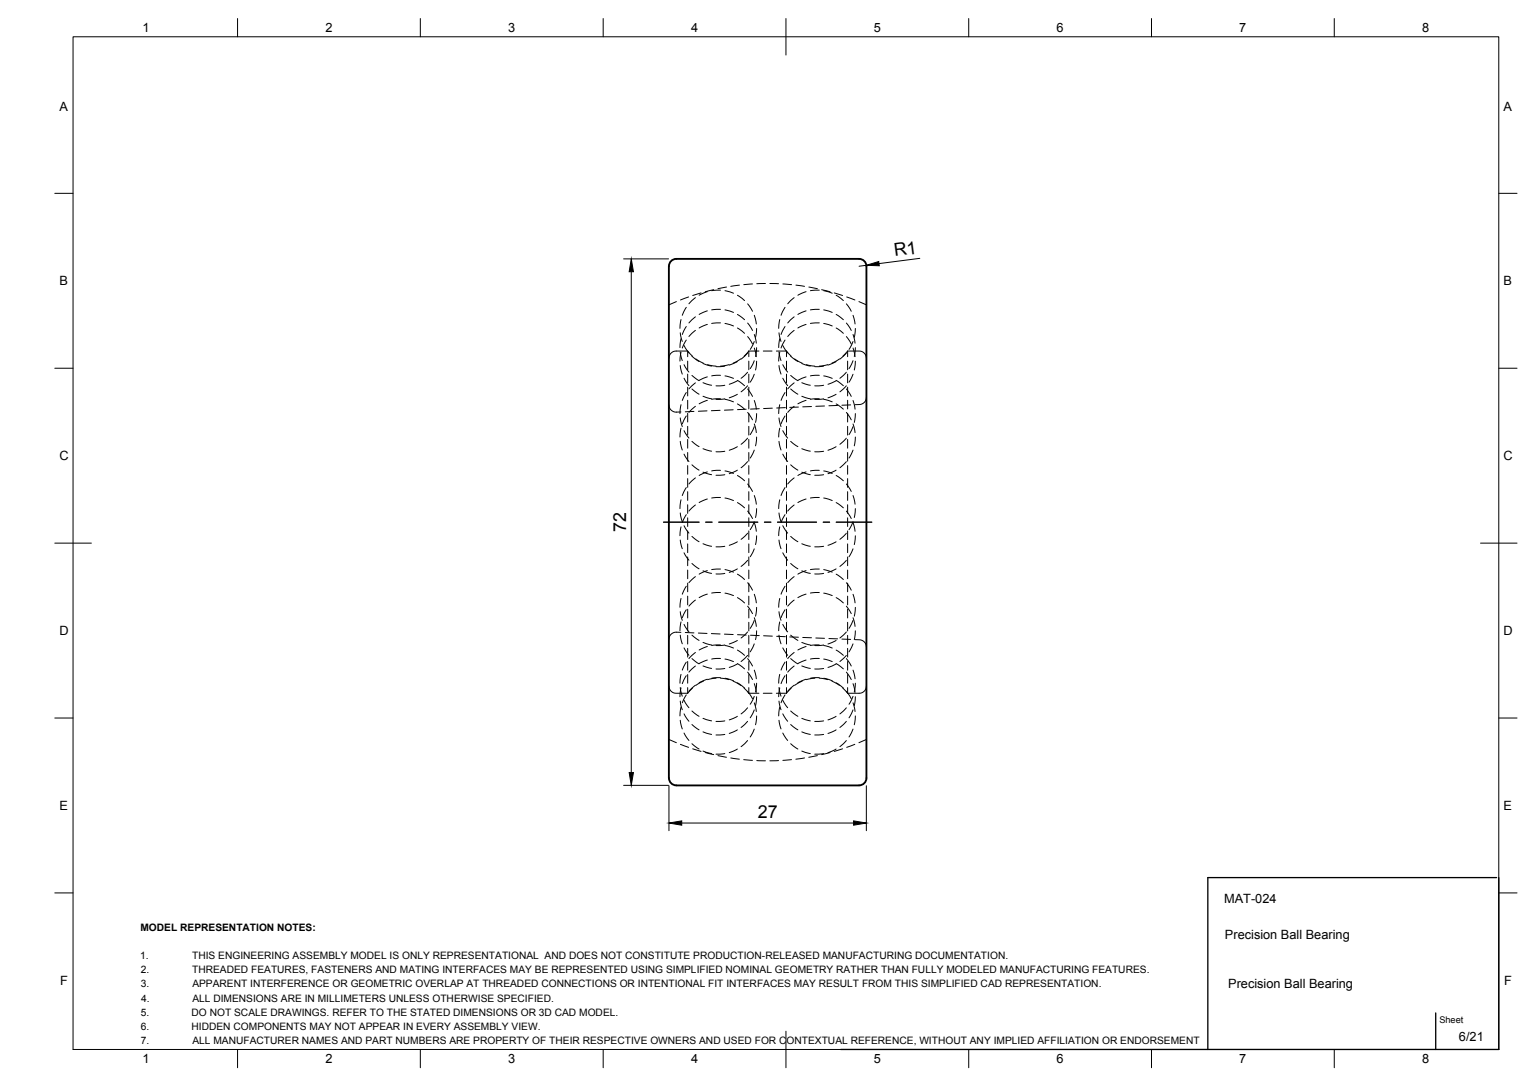
ISO-10303-21;
HEADER;
/* Generated by software containing ST-Developer
 * from STEP Tools, Inc. (www.steptools.com) 
 */

FILE_DESCRIPTION(
/* description */ ('STEP AP214'),
/* implementation_level */ '2;1');

FILE_NAME(
/* name */ 'Precision Ball Bearing.step',
/* time_stamp */ '2026-11-14T06:34:07-08:00',
/* author */ (''),
/* organization */ (''),
/* preprocessor_version */ 'ST-DEVELOPER v20.2',
/* originating_system */ 'Autodesk Translation Framework v15.17.0.0',
/* authorisation */ '');

FILE_SCHEMA (('AUTOMOTIVE_DESIGN { 1 0 10303 214 3 1 1 }'));
ENDSEC;

DATA;
#10=MECHANICAL_DESIGN_GEOMETRIC_PRESENTATION_REPRESENTATION('',(#7287,#7288,#7289,#7290,#7291,#7292,#7293,#7294,#7295,#7296,#7297,#7298,#7299,#7300,#7301,#7302,#7303,#7304,#7305,#7306,#7307,#7308,#7309,#7310,#7311,#7312),#310623);
#1040=SPHERICAL_SURFACE('',#104160,32.6421664440783);
#1041=SPHERICAL_SURFACE('',#104175,5.238);
#1042=SPHERICAL_SURFACE('',#104177,5.238);
#1043=SPHERICAL_SURFACE('',#104179,5.238);
#1044=SPHERICAL_SURFACE('',#104181,5.238);
#1045=SPHERICAL_SURFACE('',#104183,5.238);
#1046=SPHERICAL_SURFACE('',#104185,5.238);
#1047=SPHERICAL_SURFACE('',#104187,5.238);
#1048=SPHERICAL_SURFACE('',#104189,5.238);
#1049=SPHERICAL_SURFACE('',#104191,5.238);
#1050=SPHERICAL_SURFACE('',#104193,5.238);
#1051=SPHERICAL_SURFACE('',#104195,5.238);
#1052=SPHERICAL_SURFACE('',#104197,5.238);
#1053=SPHERICAL_SURFACE('',#104199,5.238);
#1054=SPHERICAL_SURFACE('',#104201,5.238);
#1055=SPHERICAL_SURFACE('',#104203,5.238);
#1056=SPHERICAL_SURFACE('',#104205,5.238);
#1057=SPHERICAL_SURFACE('',#104207,5.238);
#1058=SPHERICAL_SURFACE('',#104209,5.238);
#1059=SPHERICAL_SURFACE('',#104211,5.238);
#1060=SPHERICAL_SURFACE('',#104213,5.238);
#1061=SPHERICAL_SURFACE('',#104215,5.238);
#1062=SPHERICAL_SURFACE('',#104217,5.238);
#1063=SPHERICAL_SURFACE('',#104219,5.238);
#1064=SPHERICAL_SURFACE('',#104221,5.238);
#4116=TOROIDAL_SURFACE('',#104130,16.0425342723895,1.);
#4117=TOROIDAL_SURFACE('',#104134,26.5598538869239,5.238);
#4118=TOROIDAL_SURFACE('',#104138,26.5598538869239,5.238);
#4119=TOROIDAL_SURFACE('',#104144,17.0841991774145,1.);
#4120=TOROIDAL_SURFACE('',#104147,22.4,1.);
#4121=TOROIDAL_SURFACE('',#104155,22.4,1.);
#4122=TOROIDAL_SURFACE('',#104164,35.,1.);
#4123=TOROIDAL_SURFACE('',#104170,35.,1.);
#7163=CONICAL_SURFACE('',#104142,16.0850661013937,0.0416425087550466);
#7230=SHAPE_REPRESENTATION_RELATIONSHIP('SRR','None',#310903,#7247);
#7247=ADVANCED_BREP_SHAPE_REPRESENTATION('',(#7355,#7356,#7357,#7358,#7359,
#7360,#7361,#7362,#7363,#7364,#7365,#7366,#7367,#7368,#7369,#7370,#7371,
#7372,#7373,#7374,#7375,#7376,#7377,#7378,#7379,#7380),#310612);
#7287=STYLED_ITEM('',(#311007),#7355);
#7288=STYLED_ITEM('',(#311007),#7356);
#7289=STYLED_ITEM('',(#311007),#7357);
#7290=STYLED_ITEM('',(#311007),#7358);
#7291=STYLED_ITEM('',(#311007),#7359);
#7292=STYLED_ITEM('',(#311007),#7360);
#7293=STYLED_ITEM('',(#311007),#7361);
#7294=STYLED_ITEM('',(#311007),#7362);
#7295=STYLED_ITEM('',(#311007),#7363);
#7296=STYLED_ITEM('',(#311007),#7364);
#7297=STYLED_ITEM('',(#311007),#7365);
#7298=STYLED_ITEM('',(#311007),#7366);
#7299=STYLED_ITEM('',(#311007),#7367);
#7300=STYLED_ITEM('',(#311007),#7368);
#7301=STYLED_ITEM('',(#311007),#7369);
#7302=STYLED_ITEM('',(#311007),#7370);
#7303=STYLED_ITEM('',(#311007),#7371);
#7304=STYLED_ITEM('',(#311007),#7372);
#7305=STYLED_ITEM('',(#311007),#7373);
#7306=STYLED_ITEM('',(#311007),#7374);
#7307=STYLED_ITEM('',(#311007),#7375);
#7308=STYLED_ITEM('',(#311007),#7376);
#7309=STYLED_ITEM('',(#311007),#7377);
#7310=STYLED_ITEM('',(#311007),#7378);
#7311=STYLED_ITEM('',(#311007),#7379);
#7312=STYLED_ITEM('',(#311007),#7380);
#7355=MANIFOLD_SOLID_BREP('Body1',#93737);
#7356=MANIFOLD_SOLID_BREP('Body2',#93738);
#7357=MANIFOLD_SOLID_BREP('Body3',#93739);
#7358=MANIFOLD_SOLID_BREP('Body4',#93740);
#7359=MANIFOLD_SOLID_BREP('Body5',#93741);
#7360=MANIFOLD_SOLID_BREP('Body6',#93742);
#7361=MANIFOLD_SOLID_BREP('Body7',#93743);
#7362=MANIFOLD_SOLID_BREP('Body8',#93744);
#7363=MANIFOLD_SOLID_BREP('Body9',#93745);
#7364=MANIFOLD_SOLID_BREP('Body10',#93746);
#7365=MANIFOLD_SOLID_BREP('Body11',#93747);
#7366=MANIFOLD_SOLID_BREP('Body12',#93748);
#7367=MANIFOLD_SOLID_BREP('Body13',#93749);
#7368=MANIFOLD_SOLID_BREP('Body14',#93750);
#7369=MANIFOLD_SOLID_BREP('Body15',#93751);
#7370=MANIFOLD_SOLID_BREP('Body16',#93752);
#7371=MANIFOLD_SOLID_BREP('Body17',#93753);
#7372=MANIFOLD_SOLID_BREP('Body18',#93754);
#7373=MANIFOLD_SOLID_BREP('Body19',#93755);
#7374=MANIFOLD_SOLID_BREP('Body20',#93756);
#7375=MANIFOLD_SOLID_BREP('Body21',#93757);
#7376=MANIFOLD_SOLID_BREP('Body22',#93758);
#7377=MANIFOLD_SOLID_BREP('Body23',#93759);
#7378=MANIFOLD_SOLID_BREP('Body24',#93760);
#7379=MANIFOLD_SOLID_BREP('Body25',#93761);
#7380=MANIFOLD_SOLID_BREP('Body26',#93762);
#7642=FACE_BOUND('',#19961,.T.);
#7643=FACE_BOUND('',#19963,.T.);
#7644=FACE_BOUND('',#19965,.T.);
#7645=FACE_BOUND('',#19966,.T.);
#7646=FACE_BOUND('',#19971,.T.);
#7647=FACE_BOUND('',#19973,.T.);
#8553=PLANE('',#104158);
#8554=PLANE('',#104159);
#8555=PLANE('',#104173);
#8556=PLANE('',#104174);
#13960=FACE_OUTER_BOUND('',#19950,.T.);
#13961=FACE_OUTER_BOUND('',#19951,.T.);
#13962=FACE_OUTER_BOUND('',#19952,.T.);
#13963=FACE_OUTER_BOUND('',#19953,.T.);
#13964=FACE_OUTER_BOUND('',#19954,.T.);
#13965=FACE_OUTER_BOUND('',#19955,.T.);
#13966=FACE_OUTER_BOUND('',#19956,.T.);
#13967=FACE_OUTER_BOUND('',#19957,.T.);
#13968=FACE_OUTER_BOUND('',#19958,.T.);
#13969=FACE_OUTER_BOUND('',#19959,.T.);
#13970=FACE_OUTER_BOUND('',#19960,.T.);
#13971=FACE_OUTER_BOUND('',#19962,.T.);
#13972=FACE_OUTER_BOUND('',#19964,.T.);
#13973=FACE_OUTER_BOUND('',#19967,.T.);
#13974=FACE_OUTER_BOUND('',#19968,.T.);
#13975=FACE_OUTER_BOUND('',#19969,.T.);
#13976=FACE_OUTER_BOUND('',#19970,.T.);
#13977=FACE_OUTER_BOUND('',#19972,.T.);
#13978=FACE_OUTER_BOUND('',#19974,.T.);
#13979=FACE_OUTER_BOUND('',#19975,.T.);
#13980=FACE_OUTER_BOUND('',#19976,.T.);
#13981=FACE_OUTER_BOUND('',#19977,.T.);
#13982=FACE_OUTER_BOUND('',#19978,.T.);
#13983=FACE_OUTER_BOUND('',#19979,.T.);
#13984=FACE_OUTER_BOUND('',#19980,.T.);
#13985=FACE_OUTER_BOUND('',#19981,.T.);
#13986=FACE_OUTER_BOUND('',#19982,.T.);
#13987=FACE_OUTER_BOUND('',#19983,.T.);
#13988=FACE_OUTER_BOUND('',#19984,.T.);
#13989=FACE_OUTER_BOUND('',#19985,.T.);
#13990=FACE_OUTER_BOUND('',#19986,.T.);
#13991=FACE_OUTER_BOUND('',#19987,.T.);
#13992=FACE_OUTER_BOUND('',#19988,.T.);
#13993=FACE_OUTER_BOUND('',#19989,.T.);
#13994=FACE_OUTER_BOUND('',#19990,.T.);
#13995=FACE_OUTER_BOUND('',#19991,.T.);
#13996=FACE_OUTER_BOUND('',#19992,.T.);
#13997=FACE_OUTER_BOUND('',#19993,.T.);
#13998=FACE_OUTER_BOUND('',#19994,.T.);
#13999=FACE_OUTER_BOUND('',#19995,.T.);
#14000=FACE_OUTER_BOUND('',#19996,.T.);
#14001=FACE_OUTER_BOUND('',#19997,.T.);
#19950=EDGE_LOOP('',(#83543,#83544,#83545,#83546));
#19951=EDGE_LOOP('',(#83547,#83548,#83549,#83550));
#19952=EDGE_LOOP('',(#83551,#83552,#83553,#83554));
#19953=EDGE_LOOP('',(#83555,#83556,#83557,#83558));
#19954=EDGE_LOOP('',(#83559,#83560,#83561,#83562));
#19955=EDGE_LOOP('',(#83563,#83564,#83565,#83566));
#19956=EDGE_LOOP('',(#83567,#83568,#83569,#83570));
#19957=EDGE_LOOP('',(#83571,#83572,#83573,#83574));
#19958=EDGE_LOOP('',(#83575,#83576,#83577,#83578));
#19959=EDGE_LOOP('',(#83579,#83580,#83581,#83582));
#19960=EDGE_LOOP('',(#83583));
#19961=EDGE_LOOP('',(#83584));
#19962=EDGE_LOOP('',(#83585));
#19963=EDGE_LOOP('',(#83586));
#19964=EDGE_LOOP('',(#83587,#83588));
#19965=EDGE_LOOP('',(#83589));
#19966=EDGE_LOOP('',(#83590));
#19967=EDGE_LOOP('',(#83591,#83592,#83593,#83594));
#19968=EDGE_LOOP('',(#83595,#83596,#83597,#83598));
#19969=EDGE_LOOP('',(#83599,#83600,#83601,#83602));
#19970=EDGE_LOOP('',(#83603));
#19971=EDGE_LOOP('',(#83604));
#19972=EDGE_LOOP('',(#83605));
#19973=EDGE_LOOP('',(#83606));
#19974=EDGE_LOOP('',(#83607,#83608));
#19975=EDGE_LOOP('',(#83609,#83610));
#19976=EDGE_LOOP('',(#83611,#83612));
#19977=EDGE_LOOP('',(#83613,#83614));
#19978=EDGE_LOOP('',(#83615,#83616));
#19979=EDGE_LOOP('',(#83617,#83618));
#19980=EDGE_LOOP('',(#83619,#83620));
#19981=EDGE_LOOP('',(#83621,#83622));
#19982=EDGE_LOOP('',(#83623,#83624));
#19983=EDGE_LOOP('',(#83625,#83626));
#19984=EDGE_LOOP('',(#83627,#83628));
#19985=EDGE_LOOP('',(#83629,#83630));
#19986=EDGE_LOOP('',(#83631,#83632));
#19987=EDGE_LOOP('',(#83633,#83634));
#19988=EDGE_LOOP('',(#83635,#83636));
#19989=EDGE_LOOP('',(#83637,#83638));
#19990=EDGE_LOOP('',(#83639,#83640));
#19991=EDGE_LOOP('',(#83641,#83642));
#19992=EDGE_LOOP('',(#83643,#83644));
#19993=EDGE_LOOP('',(#83645,#83646));
#19994=EDGE_LOOP('',(#83647,#83648));
#19995=EDGE_LOOP('',(#83649,#83650));
#19996=EDGE_LOOP('',(#83651,#83652));
#19997=EDGE_LOOP('',(#83653,#83654));
#24435=LINE('',#275346,#28782);
#24436=LINE('',#275359,#28783);
#24437=LINE('',#275361,#28784);
#24438=LINE('',#275364,#28785);
#24439=LINE('',#275388,#28786);
#28782=VECTOR('',#129178,16.0850661013937);
#28783=VECTOR('',#129197,23.4);
#28784=VECTOR('',#129200,23.4);
#28785=VECTOR('',#129203,23.4);
#28786=VECTOR('',#129234,36.);
#34887=CIRCLE('',#104131,16.0425342723895);
#34888=CIRCLE('',#104132,1.);
#34889=CIRCLE('',#104133,15.0434011963687);
#34890=CIRCLE('',#104135,23.4);
#34891=CIRCLE('',#104136,5.238);
#34892=CIRCLE('',#104137,23.4);
#34893=CIRCLE('',#104139,23.4);
#34894=CIRCLE('',#104140,5.238);
#34895=CIRCLE('',#104141,23.4);
#34896=CIRCLE('',#104143,16.0850661013937);
#34897=CIRCLE('',#104145,1.);
#34898=CIRCLE('',#104146,17.0841991774145);
#34899=CIRCLE('',#104148,22.4);
#34900=CIRCLE('',#104149,1.);
#34901=CIRCLE('',#104150,23.4);
#34902=CIRCLE('',#104154,23.4);
#34903=CIRCLE('',#104156,1.);
#34904=CIRCLE('',#104157,22.4);
#34905=CIRCLE('',#104161,32.6421664440783);
#34906=CIRCLE('',#104162,29.7197077738478);
#34907=CIRCLE('',#104163,29.7197077738479);
#34908=CIRCLE('',#104165,35.);
#34909=CIRCLE('',#104166,1.);
#34910=CIRCLE('',#104167,36.);
#34911=CIRCLE('',#104169,36.);
#34912=CIRCLE('',#104171,1.);
#34913=CIRCLE('',#104172,35.);
#34914=CIRCLE('',#104176,5.238);
#34915=CIRCLE('',#104178,5.238);
#34916=CIRCLE('',#104180,5.238);
#34917=CIRCLE('',#104182,5.238);
#34918=CIRCLE('',#104184,5.238);
#34919=CIRCLE('',#104186,5.238);
#34920=CIRCLE('',#104188,5.238);
#34921=CIRCLE('',#104190,5.238);
#34922=CIRCLE('',#104192,5.238);
#34923=CIRCLE('',#104194,5.238);
#34924=CIRCLE('',#104196,5.238);
#34925=CIRCLE('',#104198,5.238);
#34926=CIRCLE('',#104200,5.238);
#34927=CIRCLE('',#104202,5.238);
#34928=CIRCLE('',#104204,5.238);
#34929=CIRCLE('',#104206,5.238);
#34930=CIRCLE('',#104208,5.238);
#34931=CIRCLE('',#104210,5.238);
#34932=CIRCLE('',#104212,5.238);
#34933=CIRCLE('',#104214,5.238);
#34934=CIRCLE('',#104216,5.238);
#34935=CIRCLE('',#104218,5.238);
#34936=CIRCLE('',#104220,5.238);
#34937=CIRCLE('',#104222,5.238);
#42861=VERTEX_POINT('',#275327);
#42862=VERTEX_POINT('',#275329);
#42863=VERTEX_POINT('',#275333);
#42864=VERTEX_POINT('',#275335);
#42865=VERTEX_POINT('',#275339);
#42866=VERTEX_POINT('',#275341);
#42867=VERTEX_POINT('',#275345);
#42868=VERTEX_POINT('',#275349);
#42869=VERTEX_POINT('',#275353);
#42870=VERTEX_POINT('',#275355);
#42871=VERTEX_POINT('',#275363);
#42872=VERTEX_POINT('',#275367);
#42873=VERTEX_POINT('',#275373);
#42874=VERTEX_POINT('',#275374);
#42875=VERTEX_POINT('',#275376);
#42876=VERTEX_POINT('',#275378);
#42877=VERTEX_POINT('',#275381);
#42878=VERTEX_POINT('',#275383);
#42879=VERTEX_POINT('',#275387);
#42880=VERTEX_POINT('',#275391);
#42881=VERTEX_POINT('',#275397);
#42882=VERTEX_POINT('',#275398);
#42883=VERTEX_POINT('',#275401);
#42884=VERTEX_POINT('',#275402);
#42885=VERTEX_POINT('',#275405);
#42886=VERTEX_POINT('',#275406);
#42887=VERTEX_POINT('',#275409);
#42888=VERTEX_POINT('',#275410);
#42889=VERTEX_POINT('',#275413);
#42890=VERTEX_POINT('',#275414);
#42891=VERTEX_POINT('',#275417);
#42892=VERTEX_POINT('',#275418);
#42893=VERTEX_POINT('',#275421);
#42894=VERTEX_POINT('',#275422);
#42895=VERTEX_POINT('',#275425);
#42896=VERTEX_POINT('',#275426);
#42897=VERTEX_POINT('',#275429);
#42898=VERTEX_POINT('',#275430);
#42899=VERTEX_POINT('',#275433);
#42900=VERTEX_POINT('',#275434);
#42901=VERTEX_POINT('',#275437);
#42902=VERTEX_POINT('',#275438);
#42903=VERTEX_POINT('',#275441);
#42904=VERTEX_POINT('',#275442);
#42905=VERTEX_POINT('',#275445);
#42906=VERTEX_POINT('',#275446);
#42907=VERTEX_POINT('',#275449);
#42908=VERTEX_POINT('',#275450);
#42909=VERTEX_POINT('',#275453);
#42910=VERTEX_POINT('',#275454);
#42911=VERTEX_POINT('',#275457);
#42912=VERTEX_POINT('',#275458);
#42913=VERTEX_POINT('',#275461);
#42914=VERTEX_POINT('',#275462);
#42915=VERTEX_POINT('',#275465);
#42916=VERTEX_POINT('',#275466);
#42917=VERTEX_POINT('',#275469);
#42918=VERTEX_POINT('',#275470);
#42919=VERTEX_POINT('',#275473);
#42920=VERTEX_POINT('',#275474);
#42921=VERTEX_POINT('',#275477);
#42922=VERTEX_POINT('',#275478);
#42923=VERTEX_POINT('',#275481);
#42924=VERTEX_POINT('',#275482);
#42925=VERTEX_POINT('',#275485);
#42926=VERTEX_POINT('',#275486);
#42927=VERTEX_POINT('',#275489);
#42928=VERTEX_POINT('',#275490);
#56551=EDGE_CURVE('',#42861,#42861,#34887,.T.);
#56552=EDGE_CURVE('',#42861,#42862,#34888,.T.);
#56553=EDGE_CURVE('',#42862,#42862,#34889,.T.);
#56554=EDGE_CURVE('',#42863,#42863,#34890,.T.);
#56555=EDGE_CURVE('',#42863,#42864,#34891,.T.);
#56556=EDGE_CURVE('',#42864,#42864,#34892,.T.);
#56557=EDGE_CURVE('',#42865,#42865,#34893,.T.);
#56558=EDGE_CURVE('',#42865,#42866,#34894,.T.);
#56559=EDGE_CURVE('',#42866,#42866,#34895,.T.);
#56560=EDGE_CURVE('',#42862,#42867,#24435,.T.);
#56561=EDGE_CURVE('',#42867,#42867,#34896,.T.);
#56562=EDGE_CURVE('',#42867,#42868,#34897,.T.);
#56563=EDGE_CURVE('',#42868,#42868,#34898,.T.);
#56564=EDGE_CURVE('',#42869,#42869,#34899,.T.);
#56565=EDGE_CURVE('',#42869,#42870,#34900,.T.);
#56566=EDGE_CURVE('',#42870,#42870,#34901,.T.);
#56567=EDGE_CURVE('',#42870,#42863,#24436,.T.);
#56568=EDGE_CURVE('',#42864,#42865,#24437,.T.);
#56569=EDGE_CURVE('',#42866,#42871,#24438,.T.);
#56570=EDGE_CURVE('',#42871,#42871,#34902,.T.);
#56571=EDGE_CURVE('',#42871,#42872,#34903,.T.);
#56572=EDGE_CURVE('',#42872,#42872,#34904,.T.);
#56573=EDGE_CURVE('',#42873,#42874,#34905,.T.);
#56574=EDGE_CURVE('',#42875,#42875,#34906,.T.);
#56575=EDGE_CURVE('',#42876,#42876,#34907,.T.);
#56576=EDGE_CURVE('',#42877,#42877,#34908,.T.);
#56577=EDGE_CURVE('',#42877,#42878,#34909,.T.);
#56578=EDGE_CURVE('',#42878,#42878,#34910,.T.);
#56579=EDGE_CURVE('',#42878,#42879,#24439,.T.);
#56580=EDGE_CURVE('',#42879,#42879,#34911,.T.);
#56581=EDGE_CURVE('',#42879,#42880,#34912,.T.);
#56582=EDGE_CURVE('',#42880,#42880,#34913,.T.);
#56583=EDGE_CURVE('',#42881,#42882,#34914,.T.);
#56584=EDGE_CURVE('',#42883,#42884,#34915,.T.);
#56585=EDGE_CURVE('',#42885,#42886,#34916,.T.);
#56586=EDGE_CURVE('',#42887,#42888,#34917,.T.);
#56587=EDGE_CURVE('',#42889,#42890,#34918,.T.);
#56588=EDGE_CURVE('',#42891,#42892,#34919,.T.);
#56589=EDGE_CURVE('',#42893,#42894,#34920,.T.);
#56590=EDGE_CURVE('',#42895,#42896,#34921,.T.);
#56591=EDGE_CURVE('',#42897,#42898,#34922,.T.);
#56592=EDGE_CURVE('',#42899,#42900,#34923,.T.);
#56593=EDGE_CURVE('',#42901,#42902,#34924,.T.);
#56594=EDGE_CURVE('',#42903,#42904,#34925,.T.);
#56595=EDGE_CURVE('',#42905,#42906,#34926,.T.);
#56596=EDGE_CURVE('',#42907,#42908,#34927,.T.);
#56597=EDGE_CURVE('',#42909,#42910,#34928,.T.);
#56598=EDGE_CURVE('',#42911,#42912,#34929,.T.);
#56599=EDGE_CURVE('',#42913,#42914,#34930,.T.);
#56600=EDGE_CURVE('',#42915,#42916,#34931,.T.);
#56601=EDGE_CURVE('',#42917,#42918,#34932,.T.);
#56602=EDGE_CURVE('',#42919,#42920,#34933,.T.);
#56603=EDGE_CURVE('',#42921,#42922,#34934,.T.);
#56604=EDGE_CURVE('',#42923,#42924,#34935,.T.);
#56605=EDGE_CURVE('',#42925,#42926,#34936,.T.);
#56606=EDGE_CURVE('',#42927,#42928,#34937,.T.);
#83543=ORIENTED_EDGE('',*,*,#56551,.F.);
#83544=ORIENTED_EDGE('',*,*,#56552,.T.);
#83545=ORIENTED_EDGE('',*,*,#56553,.T.);
#83546=ORIENTED_EDGE('',*,*,#56552,.F.);
#83547=ORIENTED_EDGE('',*,*,#56554,.F.);
#83548=ORIENTED_EDGE('',*,*,#56555,.T.);
#83549=ORIENTED_EDGE('',*,*,#56556,.T.);
#83550=ORIENTED_EDGE('',*,*,#56555,.F.);
#83551=ORIENTED_EDGE('',*,*,#56557,.F.);
#83552=ORIENTED_EDGE('',*,*,#56558,.T.);
#83553=ORIENTED_EDGE('',*,*,#56559,.T.);
#83554=ORIENTED_EDGE('',*,*,#56558,.F.);
#83555=ORIENTED_EDGE('',*,*,#56553,.F.);
#83556=ORIENTED_EDGE('',*,*,#56560,.T.);
#83557=ORIENTED_EDGE('',*,*,#56561,.T.);
#83558=ORIENTED_EDGE('',*,*,#56560,.F.);
#83559=ORIENTED_EDGE('',*,*,#56561,.F.);
#83560=ORIENTED_EDGE('',*,*,#56562,.T.);
#83561=ORIENTED_EDGE('',*,*,#56563,.T.);
#83562=ORIENTED_EDGE('',*,*,#56562,.F.);
#83563=ORIENTED_EDGE('',*,*,#56564,.F.);
#83564=ORIENTED_EDGE('',*,*,#56565,.T.);
#83565=ORIENTED_EDGE('',*,*,#56566,.T.);
#83566=ORIENTED_EDGE('',*,*,#56565,.F.);
#83567=ORIENTED_EDGE('',*,*,#56566,.F.);
#83568=ORIENTED_EDGE('',*,*,#56567,.T.);
#83569=ORIENTED_EDGE('',*,*,#56554,.T.);
#83570=ORIENTED_EDGE('',*,*,#56567,.F.);
#83571=ORIENTED_EDGE('',*,*,#56556,.F.);
#83572=ORIENTED_EDGE('',*,*,#56568,.T.);
#83573=ORIENTED_EDGE('',*,*,#56557,.T.);
#83574=ORIENTED_EDGE('',*,*,#56568,.F.);
#83575=ORIENTED_EDGE('',*,*,#56559,.F.);
#83576=ORIENTED_EDGE('',*,*,#56569,.T.);
#83577=ORIENTED_EDGE('',*,*,#56570,.T.);
#83578=ORIENTED_EDGE('',*,*,#56569,.F.);
#83579=ORIENTED_EDGE('',*,*,#56570,.F.);
#83580=ORIENTED_EDGE('',*,*,#56571,.T.);
#83581=ORIENTED_EDGE('',*,*,#56572,.T.);
#83582=ORIENTED_EDGE('',*,*,#56571,.F.);
#83583=ORIENTED_EDGE('',*,*,#56564,.T.);
#83584=ORIENTED_EDGE('',*,*,#56563,.F.);
#83585=ORIENTED_EDGE('',*,*,#56572,.F.);
#83586=ORIENTED_EDGE('',*,*,#56551,.T.);
#83587=ORIENTED_EDGE('',*,*,#56573,.T.);
#83588=ORIENTED_EDGE('',*,*,#56573,.F.);
#83589=ORIENTED_EDGE('',*,*,#56574,.F.);
#83590=ORIENTED_EDGE('',*,*,#56575,.T.);
#83591=ORIENTED_EDGE('',*,*,#56576,.F.);
#83592=ORIENTED_EDGE('',*,*,#56577,.T.);
#83593=ORIENTED_EDGE('',*,*,#56578,.T.);
#83594=ORIENTED_EDGE('',*,*,#56577,.F.);
#83595=ORIENTED_EDGE('',*,*,#56578,.F.);
#83596=ORIENTED_EDGE('',*,*,#56579,.T.);
#83597=ORIENTED_EDGE('',*,*,#56580,.T.);
#83598=ORIENTED_EDGE('',*,*,#56579,.F.);
#83599=ORIENTED_EDGE('',*,*,#56580,.F.);
#83600=ORIENTED_EDGE('',*,*,#56581,.T.);
#83601=ORIENTED_EDGE('',*,*,#56582,.T.);
#83602=ORIENTED_EDGE('',*,*,#56581,.F.);
#83603=ORIENTED_EDGE('',*,*,#56576,.T.);
#83604=ORIENTED_EDGE('',*,*,#56575,.F.);
#83605=ORIENTED_EDGE('',*,*,#56582,.F.);
#83606=ORIENTED_EDGE('',*,*,#56574,.T.);
#83607=ORIENTED_EDGE('',*,*,#56583,.T.);
#83608=ORIENTED_EDGE('',*,*,#56583,.F.);
#83609=ORIENTED_EDGE('',*,*,#56584,.T.);
#83610=ORIENTED_EDGE('',*,*,#56584,.F.);
#83611=ORIENTED_EDGE('',*,*,#56585,.T.);
#83612=ORIENTED_EDGE('',*,*,#56585,.F.);
#83613=ORIENTED_EDGE('',*,*,#56586,.T.);
#83614=ORIENTED_EDGE('',*,*,#56586,.F.);
#83615=ORIENTED_EDGE('',*,*,#56587,.T.);
#83616=ORIENTED_EDGE('',*,*,#56587,.F.);
#83617=ORIENTED_EDGE('',*,*,#56588,.T.);
#83618=ORIENTED_EDGE('',*,*,#56588,.F.);
#83619=ORIENTED_EDGE('',*,*,#56589,.T.);
#83620=ORIENTED_EDGE('',*,*,#56589,.F.);
#83621=ORIENTED_EDGE('',*,*,#56590,.T.);
#83622=ORIENTED_EDGE('',*,*,#56590,.F.);
#83623=ORIENTED_EDGE('',*,*,#56591,.T.);
#83624=ORIENTED_EDGE('',*,*,#56591,.F.);
#83625=ORIENTED_EDGE('',*,*,#56592,.T.);
#83626=ORIENTED_EDGE('',*,*,#56592,.F.);
#83627=ORIENTED_EDGE('',*,*,#56593,.T.);
#83628=ORIENTED_EDGE('',*,*,#56593,.F.);
#83629=ORIENTED_EDGE('',*,*,#56594,.T.);
#83630=ORIENTED_EDGE('',*,*,#56594,.F.);
#83631=ORIENTED_EDGE('',*,*,#56595,.T.);
#83632=ORIENTED_EDGE('',*,*,#56595,.F.);
#83633=ORIENTED_EDGE('',*,*,#56596,.T.);
#83634=ORIENTED_EDGE('',*,*,#56596,.F.);
#83635=ORIENTED_EDGE('',*,*,#56597,.T.);
#83636=ORIENTED_EDGE('',*,*,#56597,.F.);
#83637=ORIENTED_EDGE('',*,*,#56598,.T.);
#83638=ORIENTED_EDGE('',*,*,#56598,.F.);
#83639=ORIENTED_EDGE('',*,*,#56599,.T.);
#83640=ORIENTED_EDGE('',*,*,#56599,.F.);
#83641=ORIENTED_EDGE('',*,*,#56600,.T.);
#83642=ORIENTED_EDGE('',*,*,#56600,.F.);
#83643=ORIENTED_EDGE('',*,*,#56601,.T.);
#83644=ORIENTED_EDGE('',*,*,#56601,.F.);
#83645=ORIENTED_EDGE('',*,*,#56602,.T.);
#83646=ORIENTED_EDGE('',*,*,#56602,.F.);
#83647=ORIENTED_EDGE('',*,*,#56603,.T.);
#83648=ORIENTED_EDGE('',*,*,#56603,.F.);
#83649=ORIENTED_EDGE('',*,*,#56604,.T.);
#83650=ORIENTED_EDGE('',*,*,#56604,.F.);
#83651=ORIENTED_EDGE('',*,*,#56605,.T.);
#83652=ORIENTED_EDGE('',*,*,#56605,.F.);
#83653=ORIENTED_EDGE('',*,*,#56606,.T.);
#83654=ORIENTED_EDGE('',*,*,#56606,.F.);
#87779=CYLINDRICAL_SURFACE('',#104151,23.4);
#87780=CYLINDRICAL_SURFACE('',#104152,23.4);
#87781=CYLINDRICAL_SURFACE('',#104153,23.4);
#87782=CYLINDRICAL_SURFACE('',#104168,36.);
#93239=ADVANCED_FACE('',(#13960),#4116,.T.);
#93240=ADVANCED_FACE('',(#13961),#4117,.F.);
#93241=ADVANCED_FACE('',(#13962),#4118,.F.);
#93242=ADVANCED_FACE('',(#13963),#7163,.F.);
#93243=ADVANCED_FACE('',(#13964),#4119,.T.);
#93244=ADVANCED_FACE('',(#13965),#4120,.T.);
#93245=ADVANCED_FACE('',(#13966),#87779,.T.);
#93246=ADVANCED_FACE('',(#13967),#87780,.T.);
#93247=ADVANCED_FACE('',(#13968),#87781,.T.);
#93248=ADVANCED_FACE('',(#13969),#4121,.T.);
#93249=ADVANCED_FACE('',(#13970,#7642),#8553,.F.);
#93250=ADVANCED_FACE('',(#13971,#7643),#8554,.F.);
#93251=ADVANCED_FACE('',(#13972,#7644,#7645),#1040,.F.);
#93252=ADVANCED_FACE('',(#13973),#4122,.T.);
#93253=ADVANCED_FACE('',(#13974),#87782,.T.);
#93254=ADVANCED_FACE('',(#13975),#4123,.T.);
#93255=ADVANCED_FACE('',(#13976,#7646),#8555,.F.);
#93256=ADVANCED_FACE('',(#13977,#7647),#8556,.F.);
#93257=ADVANCED_FACE('',(#13978),#1041,.T.);
#93258=ADVANCED_FACE('',(#13979),#1042,.T.);
#93259=ADVANCED_FACE('',(#13980),#1043,.T.);
#93260=ADVANCED_FACE('',(#13981),#1044,.T.);
#93261=ADVANCED_FACE('',(#13982),#1045,.T.);
#93262=ADVANCED_FACE('',(#13983),#1046,.T.);
#93263=ADVANCED_FACE('',(#13984),#1047,.T.);
#93264=ADVANCED_FACE('',(#13985),#1048,.T.);
#93265=ADVANCED_FACE('',(#13986),#1049,.T.);
#93266=ADVANCED_FACE('',(#13987),#1050,.T.);
#93267=ADVANCED_FACE('',(#13988),#1051,.T.);
#93268=ADVANCED_FACE('',(#13989),#1052,.T.);
#93269=ADVANCED_FACE('',(#13990),#1053,.T.);
#93270=ADVANCED_FACE('',(#13991),#1054,.T.);
#93271=ADVANCED_FACE('',(#13992),#1055,.T.);
#93272=ADVANCED_FACE('',(#13993),#1056,.T.);
#93273=ADVANCED_FACE('',(#13994),#1057,.T.);
#93274=ADVANCED_FACE('',(#13995),#1058,.T.);
#93275=ADVANCED_FACE('',(#13996),#1059,.T.);
#93276=ADVANCED_FACE('',(#13997),#1060,.T.);
#93277=ADVANCED_FACE('',(#13998),#1061,.T.);
#93278=ADVANCED_FACE('',(#13999),#1062,.T.);
#93279=ADVANCED_FACE('',(#14000),#1063,.T.);
#93280=ADVANCED_FACE('',(#14001),#1064,.T.);
#93737=CLOSED_SHELL('',(#93239,#93240,#93241,#93242,#93243,#93244,#93245,
#93246,#93247,#93248,#93249,#93250));
#93738=CLOSED_SHELL('',(#93251,#93252,#93253,#93254,#93255,#93256));
#93739=CLOSED_SHELL('',(#93257));
#93740=CLOSED_SHELL('',(#93258));
#93741=CLOSED_SHELL('',(#93259));
#93742=CLOSED_SHELL('',(#93260));
#93743=CLOSED_SHELL('',(#93261));
#93744=CLOSED_SHELL('',(#93262));
#93745=CLOSED_SHELL('',(#93263));
#93746=CLOSED_SHELL('',(#93264));
#93747=CLOSED_SHELL('',(#93265));
#93748=CLOSED_SHELL('',(#93266));
#93749=CLOSED_SHELL('',(#93267));
#93750=CLOSED_SHELL('',(#93268));
#93751=CLOSED_SHELL('',(#93269));
#93752=CLOSED_SHELL('',(#93270));
#93753=CLOSED_SHELL('',(#93271));
#93754=CLOSED_SHELL('',(#93272));
#93755=CLOSED_SHELL('',(#93273));
#93756=CLOSED_SHELL('',(#93274));
#93757=CLOSED_SHELL('',(#93275));
#93758=CLOSED_SHELL('',(#93276));
#93759=CLOSED_SHELL('',(#93277));
#93760=CLOSED_SHELL('',(#93278));
#93761=CLOSED_SHELL('',(#93279));
#93762=CLOSED_SHELL('',(#93280));
#104129=AXIS2_PLACEMENT_3D('',#275325,#129150,#129151);
#104130=AXIS2_PLACEMENT_3D('',#275326,#129152,#129153);
#104131=AXIS2_PLACEMENT_3D('',#275328,#129154,#129155);
#104132=AXIS2_PLACEMENT_3D('',#275330,#129156,#129157);
#104133=AXIS2_PLACEMENT_3D('',#275331,#129158,#129159);
#104134=AXIS2_PLACEMENT_3D('',#275332,#129160,#129161);
#104135=AXIS2_PLACEMENT_3D('',#275334,#129162,#129163);
#104136=AXIS2_PLACEMENT_3D('',#275336,#129164,#129165);
#104137=AXIS2_PLACEMENT_3D('',#275337,#129166,#129167);
#104138=AXIS2_PLACEMENT_3D('',#275338,#129168,#129169);
#104139=AXIS2_PLACEMENT_3D('',#275340,#129170,#129171);
#104140=AXIS2_PLACEMENT_3D('',#275342,#129172,#129173);
#104141=AXIS2_PLACEMENT_3D('',#275343,#129174,#129175);
#104142=AXIS2_PLACEMENT_3D('',#275344,#129176,#129177);
#104143=AXIS2_PLACEMENT_3D('',#275347,#129179,#129180);
#104144=AXIS2_PLACEMENT_3D('',#275348,#129181,#129182);
#104145=AXIS2_PLACEMENT_3D('',#275350,#129183,#129184);
#104146=AXIS2_PLACEMENT_3D('',#275351,#129185,#129186);
#104147=AXIS2_PLACEMENT_3D('',#275352,#129187,#129188);
#104148=AXIS2_PLACEMENT_3D('',#275354,#129189,#129190);
#104149=AXIS2_PLACEMENT_3D('',#275356,#129191,#129192);
#104150=AXIS2_PLACEMENT_3D('',#275357,#129193,#129194);
#104151=AXIS2_PLACEMENT_3D('',#275358,#129195,#129196);
#104152=AXIS2_PLACEMENT_3D('',#275360,#129198,#129199);
#104153=AXIS2_PLACEMENT_3D('',#275362,#129201,#129202);
#104154=AXIS2_PLACEMENT_3D('',#275365,#129204,#129205);
#104155=AXIS2_PLACEMENT_3D('',#275366,#129206,#129207);
#104156=AXIS2_PLACEMENT_3D('',#275368,#129208,#129209);
#104157=AXIS2_PLACEMENT_3D('',#275369,#129210,#129211);
#104158=AXIS2_PLACEMENT_3D('',#275370,#129212,#129213);
#104159=AXIS2_PLACEMENT_3D('',#275371,#129214,#129215);
#104160=AXIS2_PLACEMENT_3D('',#275372,#129216,#129217);
#104161=AXIS2_PLACEMENT_3D('',#275375,#129218,#129219);
#104162=AXIS2_PLACEMENT_3D('',#275377,#129220,#129221);
#104163=AXIS2_PLACEMENT_3D('',#275379,#129222,#129223);
#104164=AXIS2_PLACEMENT_3D('',#275380,#129224,#129225);
#104165=AXIS2_PLACEMENT_3D('',#275382,#129226,#129227);
#104166=AXIS2_PLACEMENT_3D('',#275384,#129228,#129229);
#104167=AXIS2_PLACEMENT_3D('',#275385,#129230,#129231);
#104168=AXIS2_PLACEMENT_3D('',#275386,#129232,#129233);
#104169=AXIS2_PLACEMENT_3D('',#275389,#129235,#129236);
#104170=AXIS2_PLACEMENT_3D('',#275390,#129237,#129238);
#104171=AXIS2_PLACEMENT_3D('',#275392,#129239,#129240);
#104172=AXIS2_PLACEMENT_3D('',#275393,#129241,#129242);
#104173=AXIS2_PLACEMENT_3D('',#275394,#129243,#129244);
#104174=AXIS2_PLACEMENT_3D('',#275395,#129245,#129246);
#104175=AXIS2_PLACEMENT_3D('',#275396,#129247,#129248);
#104176=AXIS2_PLACEMENT_3D('',#275399,#129249,#129250);
#104177=AXIS2_PLACEMENT_3D('',#275400,#129251,#129252);
#104178=AXIS2_PLACEMENT_3D('',#275403,#129253,#129254);
#104179=AXIS2_PLACEMENT_3D('',#275404,#129255,#129256);
#104180=AXIS2_PLACEMENT_3D('',#275407,#129257,#129258);
#104181=AXIS2_PLACEMENT_3D('',#275408,#129259,#129260);
#104182=AXIS2_PLACEMENT_3D('',#275411,#129261,#129262);
#104183=AXIS2_PLACEMENT_3D('',#275412,#129263,#129264);
#104184=AXIS2_PLACEMENT_3D('',#275415,#129265,#129266);
#104185=AXIS2_PLACEMENT_3D('',#275416,#129267,#129268);
#104186=AXIS2_PLACEMENT_3D('',#275419,#129269,#129270);
#104187=AXIS2_PLACEMENT_3D('',#275420,#129271,#129272);
#104188=AXIS2_PLACEMENT_3D('',#275423,#129273,#129274);
#104189=AXIS2_PLACEMENT_3D('',#275424,#129275,#129276);
#104190=AXIS2_PLACEMENT_3D('',#275427,#129277,#129278);
#104191=AXIS2_PLACEMENT_3D('',#275428,#129279,#129280);
#104192=AXIS2_PLACEMENT_3D('',#275431,#129281,#129282);
#104193=AXIS2_PLACEMENT_3D('',#275432,#129283,#129284);
#104194=AXIS2_PLACEMENT_3D('',#275435,#129285,#129286);
#104195=AXIS2_PLACEMENT_3D('',#275436,#129287,#129288);
#104196=AXIS2_PLACEMENT_3D('',#275439,#129289,#129290);
#104197=AXIS2_PLACEMENT_3D('',#275440,#129291,#129292);
#104198=AXIS2_PLACEMENT_3D('',#275443,#129293,#129294);
#104199=AXIS2_PLACEMENT_3D('',#275444,#129295,#129296);
#104200=AXIS2_PLACEMENT_3D('',#275447,#129297,#129298);
#104201=AXIS2_PLACEMENT_3D('',#275448,#129299,#129300);
#104202=AXIS2_PLACEMENT_3D('',#275451,#129301,#129302);
#104203=AXIS2_PLACEMENT_3D('',#275452,#129303,#129304);
#104204=AXIS2_PLACEMENT_3D('',#275455,#129305,#129306);
#104205=AXIS2_PLACEMENT_3D('',#275456,#129307,#129308);
#104206=AXIS2_PLACEMENT_3D('',#275459,#129309,#129310);
#104207=AXIS2_PLACEMENT_3D('',#275460,#129311,#129312);
#104208=AXIS2_PLACEMENT_3D('',#275463,#129313,#129314);
#104209=AXIS2_PLACEMENT_3D('',#275464,#129315,#129316);
#104210=AXIS2_PLACEMENT_3D('',#275467,#129317,#129318);
#104211=AXIS2_PLACEMENT_3D('',#275468,#129319,#129320);
#104212=AXIS2_PLACEMENT_3D('',#275471,#129321,#129322);
#104213=AXIS2_PLACEMENT_3D('',#275472,#129323,#129324);
#104214=AXIS2_PLACEMENT_3D('',#275475,#129325,#129326);
#104215=AXIS2_PLACEMENT_3D('',#275476,#129327,#129328);
#104216=AXIS2_PLACEMENT_3D('',#275479,#129329,#129330);
#104217=AXIS2_PLACEMENT_3D('',#275480,#129331,#129332);
#104218=AXIS2_PLACEMENT_3D('',#275483,#129333,#129334);
#104219=AXIS2_PLACEMENT_3D('',#275484,#129335,#129336);
#104220=AXIS2_PLACEMENT_3D('',#275487,#129337,#129338);
#104221=AXIS2_PLACEMENT_3D('',#275488,#129339,#129340);
#104222=AXIS2_PLACEMENT_3D('',#275491,#129341,#129342);
#129150=DIRECTION('axis',(0.,0.,1.));
#129151=DIRECTION('refdir',(1.,0.,0.));
#129152=DIRECTION('center_axis',(0.,0.,1.));
#129153=DIRECTION('ref_axis',(1.,0.,0.));
#129154=DIRECTION('center_axis',(0.,0.,1.));
#129155=DIRECTION('ref_axis',(1.,0.,0.));
#129156=DIRECTION('center_axis',(1.22464679914735E-16,-1.,0.));
#129157=DIRECTION('ref_axis',(-1.,-1.22464679914735E-16,0.));
#129158=DIRECTION('center_axis',(0.,0.,1.));
#129159=DIRECTION('ref_axis',(1.,0.,0.));
#129160=DIRECTION('center_axis',(0.,0.,1.));
#129161=DIRECTION('ref_axis',(1.,0.,0.));
#129162=DIRECTION('center_axis',(0.,0.,1.));
#129163=DIRECTION('ref_axis',(1.,0.,0.));
#129164=DIRECTION('center_axis',(-1.22464679914735E-16,1.,0.));
#129165=DIRECTION('ref_axis',(-1.,-1.22464679914735E-16,0.));
#129166=DIRECTION('center_axis',(0.,0.,1.));
#129167=DIRECTION('ref_axis',(1.,0.,0.));
#129168=DIRECTION('center_axis',(0.,0.,1.));
#129169=DIRECTION('ref_axis',(1.,0.,0.));
#129170=DIRECTION('center_axis',(0.,0.,1.));
#129171=DIRECTION('ref_axis',(1.,0.,0.));
#129172=DIRECTION('center_axis',(-1.22464679914735E-16,1.,0.));
#129173=DIRECTION('ref_axis',(-1.,-1.22464679914735E-16,0.));
#129174=DIRECTION('center_axis',(0.,0.,1.));
#129175=DIRECTION('ref_axis',(1.,0.,0.));
#129176=DIRECTION('center_axis',(0.,0.,1.));
#129177=DIRECTION('ref_axis',(1.,0.,0.));
#129178=DIRECTION('',(-0.0416304744296221,-5.09826272572225E-18,0.999133076020789));
#129179=DIRECTION('center_axis',(0.,0.,1.));
#129180=DIRECTION('ref_axis',(1.,0.,0.));
#129181=DIRECTION('center_axis',(0.,0.,1.));
#129182=DIRECTION('ref_axis',(1.,0.,0.));
#129183=DIRECTION('center_axis',(1.22464679914735E-16,-1.,0.));
#129184=DIRECTION('ref_axis',(-1.,-1.22464679914735E-16,0.));
#129185=DIRECTION('center_axis',(0.,0.,1.));
#129186=DIRECTION('ref_axis',(1.,0.,0.));
#129187=DIRECTION('center_axis',(0.,0.,1.));
#129188=DIRECTION('ref_axis',(1.,0.,0.));
#129189=DIRECTION('center_axis',(0.,0.,1.));
#129190=DIRECTION('ref_axis',(1.,0.,0.));
#129191=DIRECTION('center_axis',(1.22464679914735E-16,-1.,0.));
#129192=DIRECTION('ref_axis',(-1.,-1.22464679914735E-16,0.));
#129193=DIRECTION('center_axis',(0.,0.,1.));
#129194=DIRECTION('ref_axis',(1.,0.,0.));
#129195=DIRECTION('center_axis',(0.,0.,1.));
#129196=DIRECTION('ref_axis',(1.,0.,0.));
#129197=DIRECTION('',(0.,0.,-1.));
#129198=DIRECTION('center_axis',(0.,0.,1.));
#129199=DIRECTION('ref_axis',(1.,0.,0.));
#129200=DIRECTION('',(0.,0.,-1.));
#129201=DIRECTION('center_axis',(0.,0.,1.));
#129202=DIRECTION('ref_axis',(1.,0.,0.));
#129203=DIRECTION('',(0.,0.,-1.));
#129204=DIRECTION('center_axis',(0.,0.,1.));
#129205=DIRECTION('ref_axis',(1.,0.,0.));
#129206=DIRECTION('center_axis',(0.,0.,1.));
#129207=DIRECTION('ref_axis',(1.,0.,0.));
#129208=DIRECTION('center_axis',(1.22464679914735E-16,-1.,0.));
#129209=DIRECTION('ref_axis',(-1.,-1.22464679914735E-16,0.));
#129210=DIRECTION('center_axis',(0.,0.,1.));
#129211=DIRECTION('ref_axis',(1.,0.,0.));
#129212=DIRECTION('center_axis',(0.,0.,-1.));
#129213=DIRECTION('ref_axis',(-1.,0.,0.));
#129214=DIRECTION('center_axis',(0.,0.,1.));
#129215=DIRECTION('ref_axis',(1.,0.,0.));
#129216=DIRECTION('center_axis',(-1.,6.12323399573677E-17,0.));
#129217=DIRECTION('ref_axis',(0.,1.,0.));
#129218=DIRECTION('center_axis',(0.,-1.22464679914735E-16,-1.));
#129219=DIRECTION('ref_axis',(0.,-1.,1.22464679914735E-16));
#129220=DIRECTION('center_axis',(0.,0.,1.));
#129221=DIRECTION('ref_axis',(1.,0.,0.));
#129222=DIRECTION('center_axis',(0.,0.,1.));
#129223=DIRECTION('ref_axis',(1.,0.,0.));
#129224=DIRECTION('center_axis',(0.,0.,1.));
#129225=DIRECTION('ref_axis',(1.,0.,0.));
#129226=DIRECTION('center_axis',(0.,0.,1.));
#129227=DIRECTION('ref_axis',(1.,0.,0.));
#129228=DIRECTION('center_axis',(1.22464679914735E-16,-1.,0.));
#129229=DIRECTION('ref_axis',(-1.,-1.22464679914735E-16,0.));
#129230=DIRECTION('center_axis',(0.,0.,1.));
#129231=DIRECTION('ref_axis',(1.,0.,0.));
#129232=DIRECTION('center_axis',(0.,0.,1.));
#129233=DIRECTION('ref_axis',(1.,0.,0.));
#129234=DIRECTION('',(0.,0.,-1.));
#129235=DIRECTION('center_axis',(0.,0.,1.));
#129236=DIRECTION('ref_axis',(1.,0.,0.));
#129237=DIRECTION('center_axis',(0.,0.,1.));
#129238=DIRECTION('ref_axis',(1.,0.,0.));
#129239=DIRECTION('center_axis',(1.22464679914735E-16,-1.,0.));
#129240=DIRECTION('ref_axis',(-1.,-1.22464679914735E-16,0.));
#129241=DIRECTION('center_axis',(0.,0.,1.));
#129242=DIRECTION('ref_axis',(1.,0.,0.));
#129243=DIRECTION('center_axis',(0.,0.,-1.));
#129244=DIRECTION('ref_axis',(-1.,0.,0.));
#129245=DIRECTION('center_axis',(0.,0.,1.));
#129246=DIRECTION('ref_axis',(1.,0.,0.));
#129247=DIRECTION('center_axis',(-1.,0.,0.));
#129248=DIRECTION('ref_axis',(0.,0.,-1.));
#129249=DIRECTION('center_axis',(0.,1.,0.));
#129250=DIRECTION('ref_axis',(0.,0.,1.));
#129251=DIRECTION('center_axis',(-1.,0.,0.));
#129252=DIRECTION('ref_axis',(0.,0.,-1.));
#129253=DIRECTION('center_axis',(0.,1.,0.));
#129254=DIRECTION('ref_axis',(0.,0.,1.));
#129255=DIRECTION('center_axis',(-0.866025403784438,-0.500000000000001,
0.));
#129256=DIRECTION('ref_axis',(0.,0.,-1.));
#129257=DIRECTION('center_axis',(-0.500000000000001,0.866025403784438,0.));
#129258=DIRECTION('ref_axis',(0.,0.,1.));
#129259=DIRECTION('center_axis',(-0.499999999999998,-0.86602540378444,0.));
#129260=DIRECTION('ref_axis',(0.,0.,-1.));
#129261=DIRECTION('center_axis',(-0.86602540378444,0.499999999999998,0.));
#129262=DIRECTION('ref_axis',(0.,0.,1.));
#129263=DIRECTION('center_axis',(3.39128835318872E-15,-1.,0.));
#129264=DIRECTION('ref_axis',(0.,0.,-1.));
#129265=DIRECTION('center_axis',(-1.,-3.49148133884313E-15,0.));
#129266=DIRECTION('ref_axis',(0.,0.,1.));
#129267=DIRECTION('center_axis',(0.500000000000004,-0.866025403784436,0.));
#129268=DIRECTION('ref_axis',(0.,0.,-1.));
#129269=DIRECTION('center_axis',(-0.866025403784436,-0.500000000000004,
0.));
#129270=DIRECTION('ref_axis',(0.,0.,1.));
#129271=DIRECTION('center_axis',(0.866025403784442,-0.499999999999995,0.));
#129272=DIRECTION('ref_axis',(0.,0.,-1.));
#129273=DIRECTION('center_axis',(-0.499999999999995,-0.866025403784442,
0.));
#129274=DIRECTION('ref_axis',(0.,0.,1.));
#129275=DIRECTION('center_axis',(1.,0.,0.));
#129276=DIRECTION('ref_axis',(0.,0.,-1.));
#129277=DIRECTION('center_axis',(0.,-1.,0.));
#129278=DIRECTION('ref_axis',(0.,0.,1.));
#129279=DIRECTION('center_axis',(0.866025403784435,0.500000000000007,0.));
#129280=DIRECTION('ref_axis',(0.,0.,-1.));
#129281=DIRECTION('center_axis',(0.500000000000007,-0.866025403784435,0.));
#129282=DIRECTION('ref_axis',(0.,0.,1.));
#129283=DIRECTION('center_axis',(0.499999999999992,0.866025403784443,0.));
#129284=DIRECTION('ref_axis',(0.,0.,-1.));
#129285=DIRECTION('center_axis',(0.866025403784443,-0.499999999999992,0.));
#129286=DIRECTION('ref_axis',(0.,0.,1.));
#129287=DIRECTION('center_axis',(-1.01738650595661E-14,1.,0.));
#129288=DIRECTION('ref_axis',(0.,0.,-1.));
#129289=DIRECTION('center_axis',(1.,1.04744440165294E-14,0.));
#129290=DIRECTION('ref_axis',(0.,0.,1.));
#129291=DIRECTION('center_axis',(-0.500000000000011,0.866025403784433,0.));
#129292=DIRECTION('ref_axis',(0.,0.,-1.));
#129293=DIRECTION('center_axis',(0.866025403784433,0.50000000000001,0.));
#129294=DIRECTION('ref_axis',(0.,0.,1.));
#129295=DIRECTION('center_axis',(-0.866025403784445,0.499999999999989,0.));
#129296=DIRECTION('ref_axis',(0.,0.,-1.));
#129297=DIRECTION('center_axis',(0.499999999999989,0.866025403784445,0.));
#129298=DIRECTION('ref_axis',(0.,0.,1.));
#129299=DIRECTION('center_axis',(-0.866025403784438,-0.500000000000001,
0.));
#129300=DIRECTION('ref_axis',(0.,0.,-1.));
#129301=DIRECTION('center_axis',(-0.500000000000001,0.866025403784438,0.));
#129302=DIRECTION('ref_axis',(0.,0.,1.));
#129303=DIRECTION('center_axis',(-0.499999999999998,-0.86602540378444,0.));
#129304=DIRECTION('ref_axis',(0.,0.,-1.));
#129305=DIRECTION('center_axis',(-0.86602540378444,0.499999999999998,0.));
#129306=DIRECTION('ref_axis',(0.,0.,1.));
#129307=DIRECTION('center_axis',(3.39128835318872E-15,-1.,0.));
#129308=DIRECTION('ref_axis',(0.,0.,-1.));
#129309=DIRECTION('center_axis',(-1.,-3.49148133884313E-15,0.));
#129310=DIRECTION('ref_axis',(0.,0.,1.));
#129311=DIRECTION('center_axis',(0.500000000000004,-0.866025403784436,0.));
#129312=DIRECTION('ref_axis',(0.,0.,-1.));
#129313=DIRECTION('center_axis',(-0.866025403784436,-0.500000000000004,
0.));
#129314=DIRECTION('ref_axis',(0.,0.,1.));
#129315=DIRECTION('center_axis',(0.866025403784442,-0.499999999999995,0.));
#129316=DIRECTION('ref_axis',(0.,0.,-1.));
#129317=DIRECTION('center_axis',(-0.499999999999995,-0.866025403784442,
0.));
#129318=DIRECTION('ref_axis',(0.,0.,1.));
#129319=DIRECTION('center_axis',(1.,0.,0.));
#129320=DIRECTION('ref_axis',(0.,0.,-1.));
#129321=DIRECTION('center_axis',(0.,-1.,0.));
#129322=DIRECTION('ref_axis',(0.,0.,1.));
#129323=DIRECTION('center_axis',(0.866025403784435,0.500000000000007,0.));
#129324=DIRECTION('ref_axis',(0.,0.,-1.));
#129325=DIRECTION('center_axis',(0.500000000000007,-0.866025403784435,0.));
#129326=DIRECTION('ref_axis',(0.,0.,1.));
#129327=DIRECTION('center_axis',(0.499999999999992,0.866025403784443,0.));
#129328=DIRECTION('ref_axis',(0.,0.,-1.));
#129329=DIRECTION('center_axis',(0.866025403784443,-0.499999999999992,0.));
#129330=DIRECTION('ref_axis',(0.,0.,1.));
#129331=DIRECTION('center_axis',(-1.01738650595661E-14,1.,0.));
#129332=DIRECTION('ref_axis',(0.,0.,-1.));
#129333=DIRECTION('center_axis',(1.,1.04744440165294E-14,0.));
#129334=DIRECTION('ref_axis',(0.,0.,1.));
#129335=DIRECTION('center_axis',(-0.500000000000011,0.866025403784433,0.));
#129336=DIRECTION('ref_axis',(0.,0.,-1.));
#129337=DIRECTION('center_axis',(0.866025403784433,0.50000000000001,0.));
#129338=DIRECTION('ref_axis',(0.,0.,1.));
#129339=DIRECTION('center_axis',(-0.866025403784445,0.499999999999989,0.));
#129340=DIRECTION('ref_axis',(0.,0.,-1.));
#129341=DIRECTION('center_axis',(0.499999999999989,0.866025403784445,0.));
#129342=DIRECTION('ref_axis',(0.,0.,1.));
#275325=CARTESIAN_POINT('',(0.,0.,0.));
#275326=CARTESIAN_POINT('Origin',(0.,0.,-12.5));
#275327=CARTESIAN_POINT('',(-16.0425342723895,-1.96464382468935E-15,-13.5));
#275328=CARTESIAN_POINT('Origin',(0.,0.,-13.5));
#275329=CARTESIAN_POINT('',(-15.0434011963687,1.90606889192839E-15,-12.4583695255704));
#275330=CARTESIAN_POINT('Origin',(-16.0425342723895,-1.96464382468935E-15,
-12.5));
#275331=CARTESIAN_POINT('Origin',(0.,0.,-12.4583695255704));
#275332=CARTESIAN_POINT('Origin',(0.,0.,6.75));
#275333=CARTESIAN_POINT('',(-23.4,2.86567351000481E-15,10.9275551957205));
#275334=CARTESIAN_POINT('Origin',(0.,0.,10.9275551957205));
#275335=CARTESIAN_POINT('',(-23.4,-2.86567351000481E-15,2.57244480427945));
#275336=CARTESIAN_POINT('Origin',(-26.5598538869239,-3.25264400484428E-15,
6.75));
#275337=CARTESIAN_POINT('Origin',(0.,0.,2.57244480427945));
#275338=CARTESIAN_POINT('Origin',(0.,0.,-6.75));
#275339=CARTESIAN_POINT('',(-23.4,2.86567351000481E-15,-2.57244480427945));
#275340=CARTESIAN_POINT('Origin',(0.,0.,-2.57244480427945));
#275341=CARTESIAN_POINT('',(-23.4,-2.86567351000481E-15,-10.9275551957205));
#275342=CARTESIAN_POINT('Origin',(-26.5598538869239,-3.25264400484428E-15,
-6.75));
#275343=CARTESIAN_POINT('Origin',(0.,0.,-10.9275551957205));
#275344=CARTESIAN_POINT('Origin',(0.,0.,12.5416304744296));
#275345=CARTESIAN_POINT('',(-16.0850661013937,-1.96985247151454E-15,12.5416304744296));
#275346=CARTESIAN_POINT('',(-16.0850661013937,-1.96985247151454E-15,12.5416304744296));
#275347=CARTESIAN_POINT('Origin',(0.,0.,12.5416304744296));
#275348=CARTESIAN_POINT('Origin',(0.,0.,12.5));
#275349=CARTESIAN_POINT('',(-17.0841991774145,-2.09221098386165E-15,13.5));
#275350=CARTESIAN_POINT('Origin',(-17.0841991774145,-2.09221098386165E-15,
12.5));
#275351=CARTESIAN_POINT('Origin',(0.,0.,13.5));
#275352=CARTESIAN_POINT('Origin',(0.,0.,12.5));
#275353=CARTESIAN_POINT('',(-22.4,-2.74320883009007E-15,13.5));
#275354=CARTESIAN_POINT('Origin',(0.,0.,13.5));
#275355=CARTESIAN_POINT('',(-23.4,-2.86567351000481E-15,12.5));
#275356=CARTESIAN_POINT('Origin',(-22.4,-2.74320883009007E-15,12.5));
#275357=CARTESIAN_POINT('Origin',(0.,0.,12.5));
#275358=CARTESIAN_POINT('Origin',(0.,0.,0.));
#275359=CARTESIAN_POINT('',(-23.4,-2.86567351000481E-15,0.));
#275360=CARTESIAN_POINT('Origin',(0.,0.,0.));
#275361=CARTESIAN_POINT('',(-23.4,-2.86567351000481E-15,0.));
#275362=CARTESIAN_POINT('Origin',(0.,0.,0.));
#275363=CARTESIAN_POINT('',(-23.4,-2.86567351000481E-15,-12.5));
#275364=CARTESIAN_POINT('',(-23.4,-2.86567351000481E-15,0.));
#275365=CARTESIAN_POINT('Origin',(0.,0.,-12.5));
#275366=CARTESIAN_POINT('Origin',(0.,0.,-12.5));
#275367=CARTESIAN_POINT('',(-22.4,-2.74320883009007E-15,-13.5));
#275368=CARTESIAN_POINT('Origin',(-22.4,-2.74320883009007E-15,-12.5));
#275369=CARTESIAN_POINT('Origin',(0.,0.,-13.5));
#275370=CARTESIAN_POINT('Origin',(0.,22.4,13.5));
#275371=CARTESIAN_POINT('Origin',(0.,22.4,-13.5));
#275372=CARTESIAN_POINT('Origin',(0.,0.,0.));
#275373=CARTESIAN_POINT('',(32.6421664440783,-1.99875623264878E-15,2.44777042258915E-31));
#275374=CARTESIAN_POINT('',(-32.6421664440783,-1.99875623264878E-15,2.44777042258915E-31));
#275375=CARTESIAN_POINT('Origin',(0.,0.,0.));
#275376=CARTESIAN_POINT('',(0.,29.7197077738478,-13.5));
#275377=CARTESIAN_POINT('Origin',(0.,0.,-13.5));
#275378=CARTESIAN_POINT('',(0.,29.7197077738479,13.5));
#275379=CARTESIAN_POINT('Origin',(0.,0.,13.5));
#275380=CARTESIAN_POINT('Origin',(0.,0.,12.5));
#275381=CARTESIAN_POINT('',(-35.,-4.28626379701574E-15,13.5));
#275382=CARTESIAN_POINT('Origin',(0.,0.,13.5));
#275383=CARTESIAN_POINT('',(-36.,-4.40872847693047E-15,12.5));
#275384=CARTESIAN_POINT('Origin',(-35.,-4.28626379701574E-15,12.5));
#275385=CARTESIAN_POINT('Origin',(0.,0.,12.5));
#275386=CARTESIAN_POINT('Origin',(0.,0.,0.));
#275387=CARTESIAN_POINT('',(-36.,-4.40872847693047E-15,-12.5));
#275388=CARTESIAN_POINT('',(-36.,-4.40872847693047E-15,0.));
#275389=CARTESIAN_POINT('Origin',(0.,0.,-12.5));
#275390=CARTESIAN_POINT('Origin',(0.,0.,-12.5));
#275391=CARTESIAN_POINT('',(-35.,-4.28626379701574E-15,-13.5));
#275392=CARTESIAN_POINT('Origin',(-35.,-4.28626379701574E-15,-12.5));
#275393=CARTESIAN_POINT('Origin',(0.,0.,-13.5));
#275394=CARTESIAN_POINT('Origin',(0.,29.7197077738479,13.5));
#275395=CARTESIAN_POINT('Origin',(0.,35.,-13.5));
#275396=CARTESIAN_POINT('Origin',(0.,26.5598538869239,6.75));
#275397=CARTESIAN_POINT('',(-5.238,26.5598538869239,6.75));
#275398=CARTESIAN_POINT('',(5.238,26.5598538869239,6.75));
#275399=CARTESIAN_POINT('Origin',(0.,26.5598538869239,6.75));
#275400=CARTESIAN_POINT('Origin',(0.,26.5598538869239,-6.75));
#275401=CARTESIAN_POINT('',(-5.238,26.5598538869239,-6.75));
#275402=CARTESIAN_POINT('',(5.238,26.5598538869239,-6.75));
#275403=CARTESIAN_POINT('Origin',(0.,26.5598538869239,-6.75));
#275404=CARTESIAN_POINT('Origin',(-13.279926943462,23.001508186879,6.75));
#275405=CARTESIAN_POINT('',(-17.8161680084849,20.382508186879,6.75));
#275406=CARTESIAN_POINT('',(-8.7436858784391,25.620508186879,6.75));
#275407=CARTESIAN_POINT('Origin',(-13.279926943462,23.001508186879,6.75));
#275408=CARTESIAN_POINT('Origin',(-23.001508186879,13.2799269434619,6.75));
#275409=CARTESIAN_POINT('',(-25.620508186879,8.74368587843902,6.75));
#275410=CARTESIAN_POINT('',(-20.382508186879,17.8161680084848,6.75));
#275411=CARTESIAN_POINT('Origin',(-23.001508186879,13.2799269434619,6.75));
#275412=CARTESIAN_POINT('Origin',(-26.5598538869239,-9.27332342085952E-14,
6.75));
#275413=CARTESIAN_POINT('',(-26.5598538869239,-5.2380000000001,6.75));
#275414=CARTESIAN_POINT('',(-26.5598538869239,5.23799999999991,6.75));
#275415=CARTESIAN_POINT('Origin',(-26.5598538869239,-9.27332342085952E-14,
6.75));
#275416=CARTESIAN_POINT('Origin',(-23.0015081868789,-13.2799269434621,6.75));
#275417=CARTESIAN_POINT('',(-20.3825081868789,-17.816168008485,6.75));
#275418=CARTESIAN_POINT('',(-25.620508186879,-8.74368587843919,6.75));
#275419=CARTESIAN_POINT('Origin',(-23.0015081868789,-13.2799269434621,6.75));
#275420=CARTESIAN_POINT('Origin',(-13.2799269434618,-23.0015081868791,6.75));
#275421=CARTESIAN_POINT('',(-8.74368587843892,-25.620508186879,6.75));
#275422=CARTESIAN_POINT('',(-17.8161680084847,-20.3825081868791,6.75));
#275423=CARTESIAN_POINT('Origin',(-13.2799269434618,-23.0015081868791,6.75));
#275424=CARTESIAN_POINT('Origin',(0.,-26.5598538869239,6.75));
#275425=CARTESIAN_POINT('',(5.238,-26.5598538869239,6.75));
#275426=CARTESIAN_POINT('',(-5.238,-26.5598538869239,6.75));
#275427=CARTESIAN_POINT('Origin',(0.,-26.5598538869239,6.75));
#275428=CARTESIAN_POINT('Origin',(13.2799269434622,-23.0015081868789,6.75));
#275429=CARTESIAN_POINT('',(17.816168008485,-20.3825081868788,6.75));
#275430=CARTESIAN_POINT('',(8.74368587843928,-25.6205081868789,6.75));
#275431=CARTESIAN_POINT('Origin',(13.2799269434622,-23.0015081868789,6.75));
#275432=CARTESIAN_POINT('Origin',(23.0015081868791,-13.2799269434618,6.75));
#275433=CARTESIAN_POINT('',(25.6205081868791,-8.74368587843884,6.75));
#275434=CARTESIAN_POINT('',(20.3825081868792,-17.8161680084847,6.75));
#275435=CARTESIAN_POINT('Origin',(23.0015081868791,-13.2799269434618,6.75));
#275436=CARTESIAN_POINT('Origin',(26.5598538869239,2.78199702625785E-13,
6.75));
#275437=CARTESIAN_POINT('',(26.5598538869239,5.23800000000028,6.75));
#275438=CARTESIAN_POINT('',(26.559853886924,-5.23799999999972,6.75));
#275439=CARTESIAN_POINT('Origin',(26.5598538869239,2.78199702625785E-13,
6.75));
#275440=CARTESIAN_POINT('Origin',(23.0015081868788,13.2799269434622,6.75));
#275441=CARTESIAN_POINT('',(20.3825081868788,17.8161680084851,6.75));
#275442=CARTESIAN_POINT('',(25.6205081868789,8.74368587843937,6.75));
#275443=CARTESIAN_POINT('Origin',(23.0015081868788,13.2799269434622,6.75));
#275444=CARTESIAN_POINT('Origin',(13.2799269434617,23.0015081868792,6.75));
#275445=CARTESIAN_POINT('',(8.74368587843875,25.6205081868791,6.75));
#275446=CARTESIAN_POINT('',(17.8161680084846,20.3825081868792,6.75));
#275447=CARTESIAN_POINT('Origin',(13.2799269434617,23.0015081868792,6.75));
#275448=CARTESIAN_POINT('Origin',(-13.279926943462,23.001508186879,-6.75));
#275449=CARTESIAN_POINT('',(-17.8161680084849,20.382508186879,-6.75));
#275450=CARTESIAN_POINT('',(-8.7436858784391,25.620508186879,-6.75));
#275451=CARTESIAN_POINT('Origin',(-13.279926943462,23.001508186879,-6.75));
#275452=CARTESIAN_POINT('Origin',(-23.001508186879,13.2799269434619,-6.75));
#275453=CARTESIAN_POINT('',(-25.620508186879,8.74368587843901,-6.75));
#275454=CARTESIAN_POINT('',(-20.382508186879,17.8161680084848,-6.75));
#275455=CARTESIAN_POINT('Origin',(-23.001508186879,13.2799269434619,-6.75));
#275456=CARTESIAN_POINT('Origin',(-26.5598538869239,-9.27332342085952E-14,
-6.75));
#275457=CARTESIAN_POINT('',(-26.5598538869239,-5.2380000000001,-6.75));
#275458=CARTESIAN_POINT('',(-26.5598538869239,5.23799999999991,-6.75));
#275459=CARTESIAN_POINT('Origin',(-26.5598538869239,-9.27332342085952E-14,
-6.75));
#275460=CARTESIAN_POINT('Origin',(-23.0015081868789,-13.2799269434621,-6.75));
#275461=CARTESIAN_POINT('',(-20.3825081868789,-17.816168008485,-6.75));
#275462=CARTESIAN_POINT('',(-25.620508186879,-8.74368587843919,-6.75));
#275463=CARTESIAN_POINT('Origin',(-23.0015081868789,-13.2799269434621,-6.75));
#275464=CARTESIAN_POINT('Origin',(-13.2799269434618,-23.0015081868791,-6.75));
#275465=CARTESIAN_POINT('',(-8.74368587843892,-25.620508186879,-6.75));
#275466=CARTESIAN_POINT('',(-17.8161680084847,-20.3825081868791,-6.75));
#275467=CARTESIAN_POINT('Origin',(-13.2799269434618,-23.0015081868791,-6.75));
#275468=CARTESIAN_POINT('Origin',(0.,-26.5598538869239,-6.75));
#275469=CARTESIAN_POINT('',(5.238,-26.5598538869239,-6.75));
#275470=CARTESIAN_POINT('',(-5.238,-26.5598538869239,-6.75));
#275471=CARTESIAN_POINT('Origin',(0.,-26.5598538869239,-6.75));
#275472=CARTESIAN_POINT('Origin',(13.2799269434622,-23.0015081868789,-6.75));
#275473=CARTESIAN_POINT('',(17.816168008485,-20.3825081868788,-6.75));
#275474=CARTESIAN_POINT('',(8.74368587843928,-25.6205081868789,-6.75));
#275475=CARTESIAN_POINT('Origin',(13.2799269434622,-23.0015081868789,-6.75));
#275476=CARTESIAN_POINT('Origin',(23.0015081868791,-13.2799269434618,-6.75));
#275477=CARTESIAN_POINT('',(25.6205081868791,-8.74368587843884,-6.75));
#275478=CARTESIAN_POINT('',(20.3825081868792,-17.8161680084847,-6.75));
#275479=CARTESIAN_POINT('Origin',(23.0015081868791,-13.2799269434618,-6.75));
#275480=CARTESIAN_POINT('Origin',(26.5598538869239,2.78199702625785E-13,
-6.75));
#275481=CARTESIAN_POINT('',(26.5598538869239,5.23800000000028,-6.75));
#275482=CARTESIAN_POINT('',(26.559853886924,-5.23799999999973,-6.75));
#275483=CARTESIAN_POINT('Origin',(26.5598538869239,2.78199702625785E-13,
-6.75));
#275484=CARTESIAN_POINT('Origin',(23.0015081868788,13.2799269434622,-6.75));
#275485=CARTESIAN_POINT('',(20.3825081868788,17.8161680084851,-6.75));
#275486=CARTESIAN_POINT('',(25.6205081868789,8.74368587843937,-6.75));
#275487=CARTESIAN_POINT('Origin',(23.0015081868788,13.2799269434622,-6.75));
#275488=CARTESIAN_POINT('Origin',(13.2799269434617,23.0015081868792,-6.75));
#275489=CARTESIAN_POINT('',(8.74368587843874,25.6205081868791,-6.75));
#275490=CARTESIAN_POINT('',(17.8161680084846,20.3825081868792,-6.75));
#275491=CARTESIAN_POINT('Origin',(13.2799269434617,23.0015081868792,-6.75));
#310590=UNCERTAINTY_MEASURE_WITH_UNIT(LENGTH_MEASURE(0.01),#310624,
'DISTANCE_ACCURACY_VALUE',
'Maximum model space distance between geometric entities at asserted c
onnectivities');
#310601=UNCERTAINTY_MEASURE_WITH_UNIT(LENGTH_MEASURE(0.01),#310624,
'DISTANCE_ACCURACY_VALUE',
'Maximum model space distance between geometric entities at asserted c
onnectivities');
#310612=(
GEOMETRIC_REPRESENTATION_CONTEXT(3)
GLOBAL_UNCERTAINTY_ASSIGNED_CONTEXT((#310590))
GLOBAL_UNIT_ASSIGNED_CONTEXT((#310624,#310626,#310627))
REPRESENTATION_CONTEXT('','3D')
);
#310623=(
GEOMETRIC_REPRESENTATION_CONTEXT(3)
GLOBAL_UNCERTAINTY_ASSIGNED_CONTEXT((#310601))
GLOBAL_UNIT_ASSIGNED_CONTEXT((#310624,#310626,#310627))
REPRESENTATION_CONTEXT('','3D')
);
#310624=(
LENGTH_UNIT()
NAMED_UNIT(*)
SI_UNIT(.MILLI.,.METRE.)
);
#310626=(
NAMED_UNIT(*)
PLANE_ANGLE_UNIT()
SI_UNIT($,.RADIAN.)
);
#310627=(
NAMED_UNIT(*)
SI_UNIT($,.STERADIAN.)
SOLID_ANGLE_UNIT()
);
#310638=SHAPE_DEFINITION_REPRESENTATION(#310797,#310903);
#310797=PRODUCT_DEFINITION_SHAPE('',$,#310925);
#310903=SHAPE_REPRESENTATION('',(#104129),#310612);
#310914=PRODUCT_DEFINITION_CONTEXT('part definition',#310979,'design');
#310925=PRODUCT_DEFINITION('Precision Ball Bearing',
'Precision Ball Bearing',#310946,#310914);
#310946=PRODUCT_DEFINITION_FORMATION('',$,#310991);
#310979=APPLICATION_CONTEXT(
'Core Data for Automotive Mechanical Design Process');
#310980=PRODUCT_CONTEXT('part definition',#310979,'mechanical');
#310991=PRODUCT('Precision Ball Bearing','Precision Ball Bearing',$,(#310980));
#311007=PRESENTATION_STYLE_ASSIGNMENT((#311014));
#311014=SURFACE_STYLE_USAGE(.BOTH.,#311021);
#311021=SURFACE_SIDE_STYLE('',(#311028));
#311028=SURFACE_STYLE_FILL_AREA(#311035);
#311035=FILL_AREA_STYLE('Opaque(122,133,145)',(#311042));
#311042=FILL_AREA_STYLE_COLOUR('Opaque(122,133,145)',#311049);
#311049=COLOUR_RGB('Opaque(122,133,145)',0.47843137254902,0.52156862745098,
0.568627450980392);
ENDSEC;
END-ISO-10303-21;
